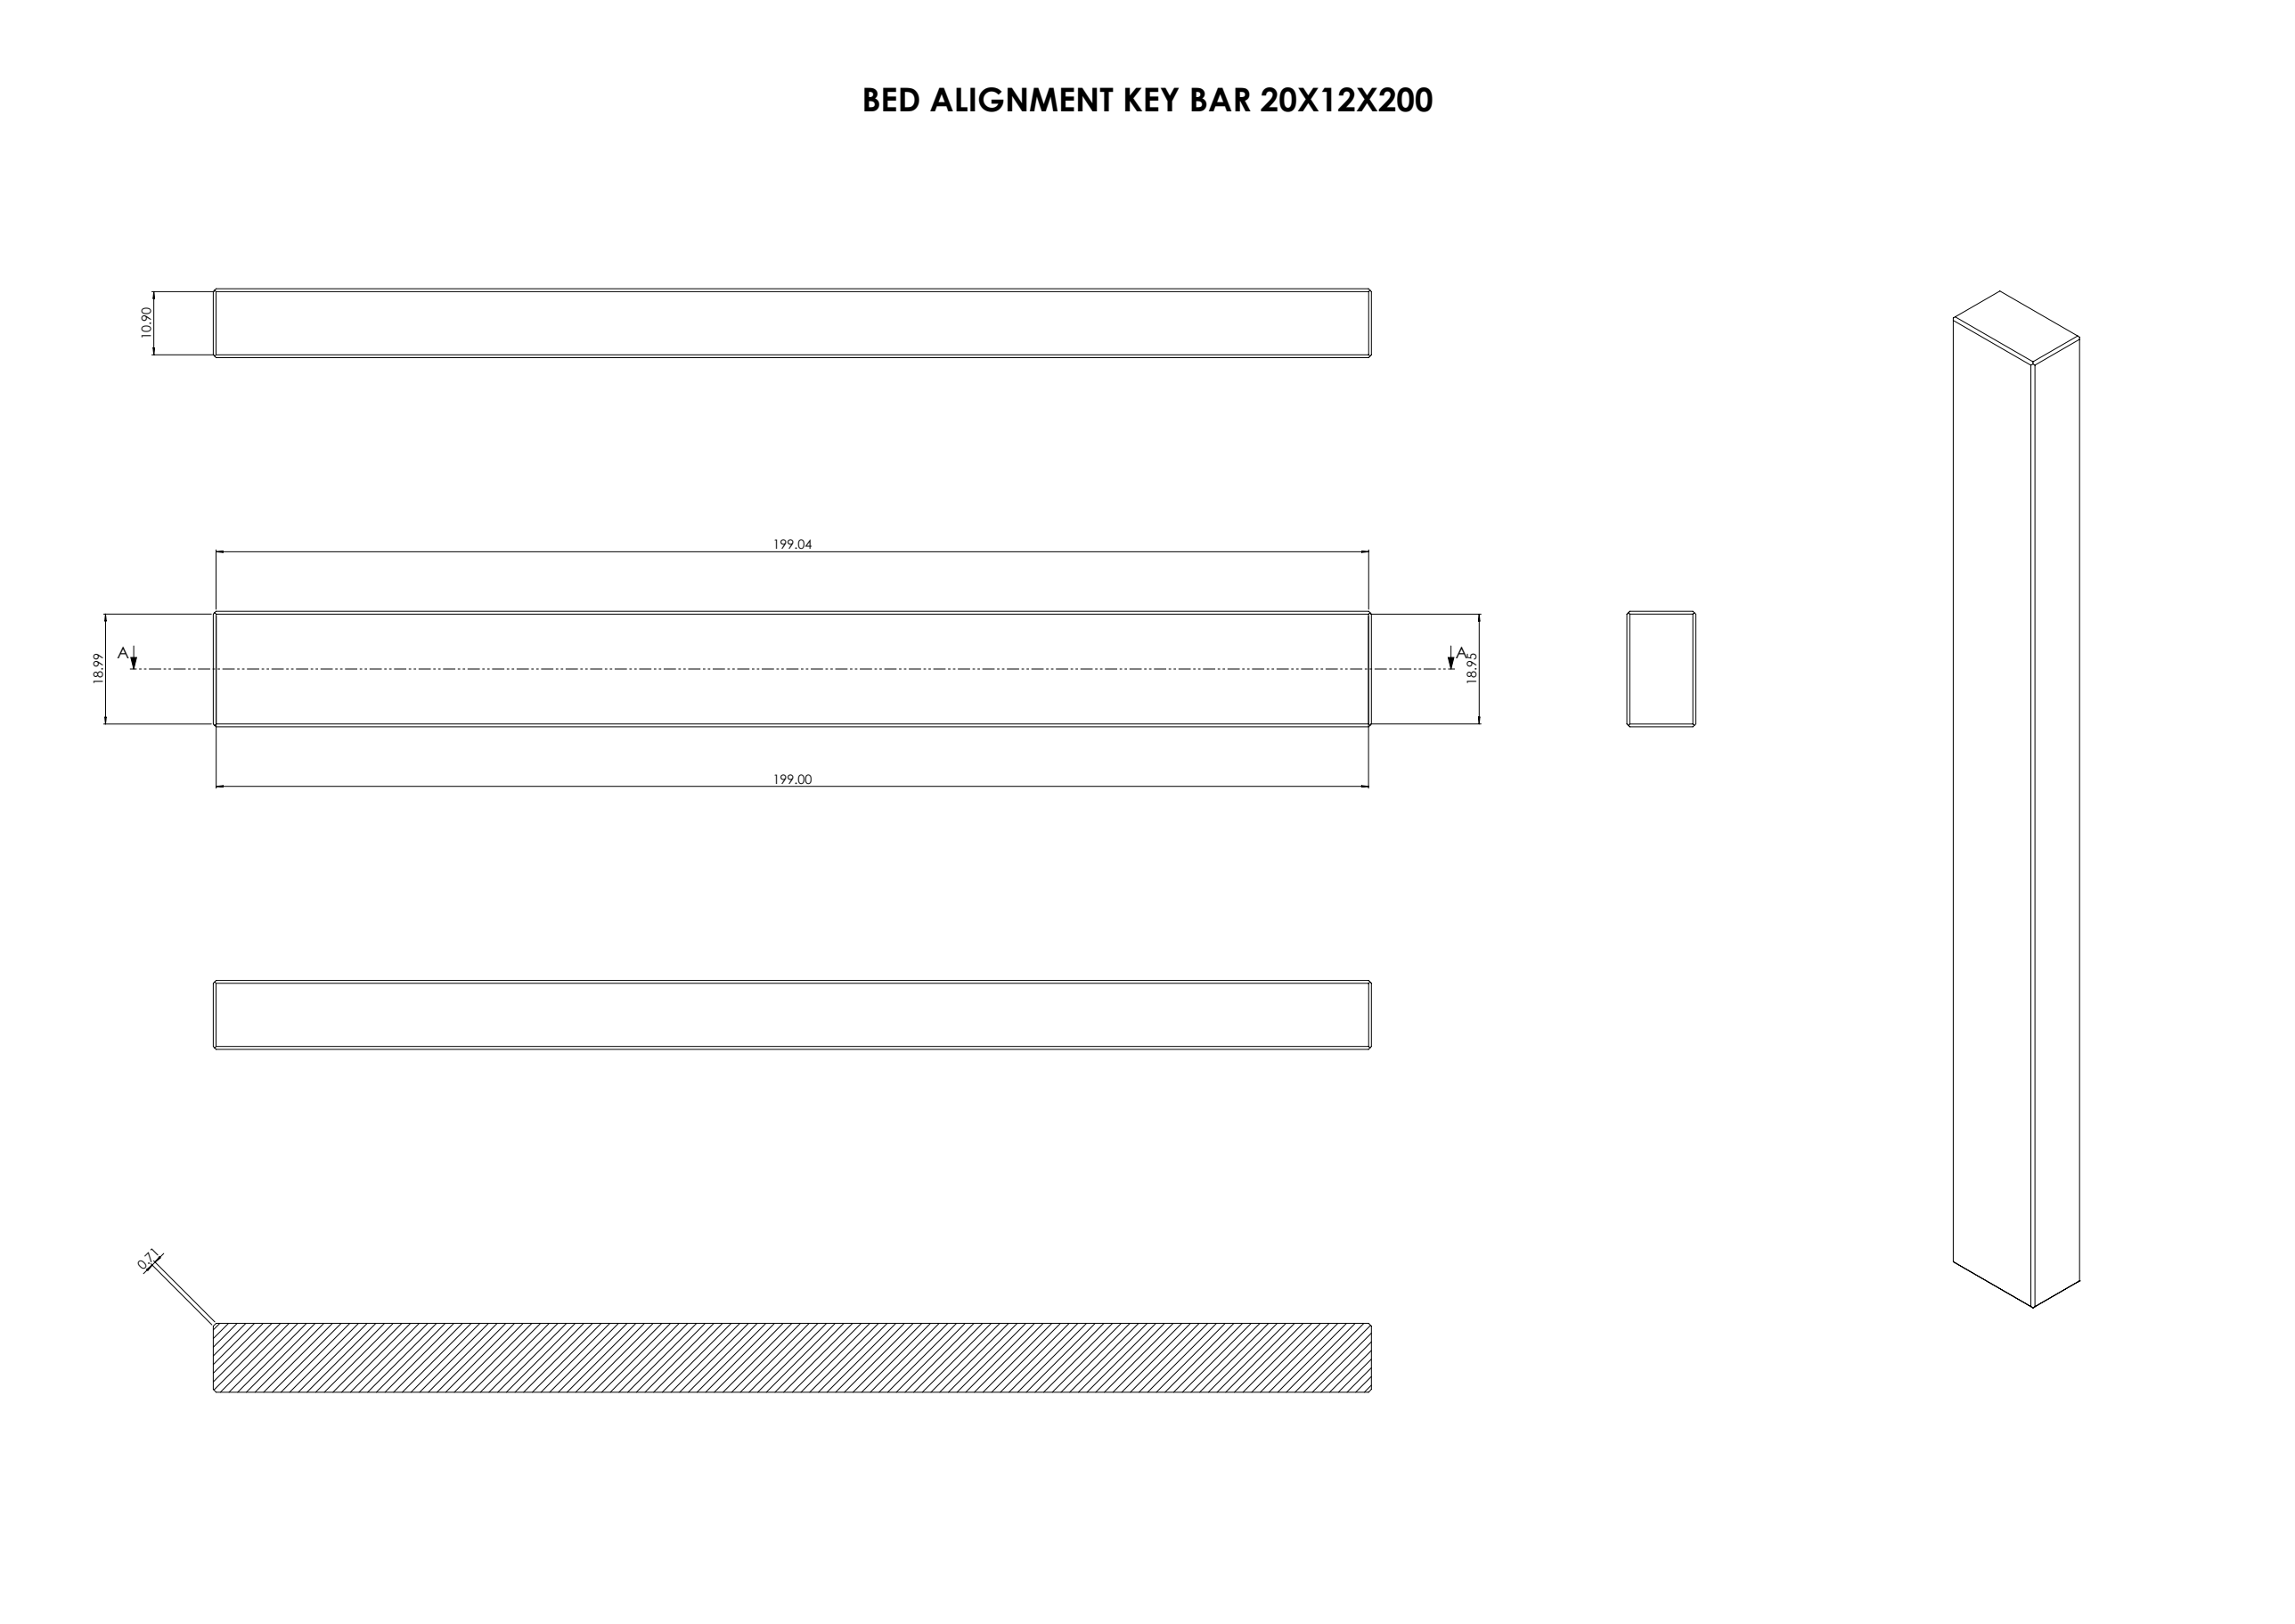
ISO-10303-21;
HEADER;
/* Generated by software containing ST-Developer
 * from STEP Tools, Inc. (www.steptools.com) 
 */

FILE_DESCRIPTION(
/* description */ (''),
/* implementation_level */ '2;1');

FILE_NAME(
/* name */ '16_Bed_Alignment_Key_Bar_20x12x200.step',
/* time_stamp */ '2026-10-26T03:50:32-07:00',
/* author */ (''),
/* organization */ (''),
/* preprocessor_version */ 'ST-DEVELOPER v20.2',
/* originating_system */ 'Autodesk Translation Framework v15.15.0.0',
/* authorisation */ '');

FILE_SCHEMA (('AUTOMOTIVE_DESIGN { 1 0 10303 214 3 1 1 }'));
ENDSEC;

DATA;
#10=MECHANICAL_DESIGN_GEOMETRIC_PRESENTATION_REPRESENTATION('',(#1052),#76660);
#1012=SHAPE_REPRESENTATION_RELATIONSHIP('SRR','None',#76749,#1032);
#1032=ADVANCED_BREP_SHAPE_REPRESENTATION('',(#1072),#76653);
#1052=STYLED_ITEM('',(#76906),#1072);
#1072=MANIFOLD_SOLID_BREP('Key bar',#26677);
#2130=PLANE('',#28345);
#2131=PLANE('',#28346);
#2132=PLANE('',#28347);
#2133=PLANE('',#28348);
#2134=PLANE('',#28349);
#2135=PLANE('',#28350);
#2136=PLANE('',#28351);
#2137=PLANE('',#28352);
#2138=PLANE('',#28353);
#2139=PLANE('',#28354);
#2140=PLANE('',#28355);
#2141=PLANE('',#28356);
#2142=PLANE('',#28357);
#2143=PLANE('',#28358);
#2144=PLANE('',#28359);
#2145=PLANE('',#28360);
#2146=PLANE('',#28361);
#2147=PLANE('',#28362);
#3436=FACE_OUTER_BOUND('',#5075,.T.);
#3437=FACE_OUTER_BOUND('',#5076,.T.);
#3438=FACE_OUTER_BOUND('',#5077,.T.);
#3439=FACE_OUTER_BOUND('',#5078,.T.);
#3440=FACE_OUTER_BOUND('',#5079,.T.);
#3441=FACE_OUTER_BOUND('',#5080,.T.);
#3442=FACE_OUTER_BOUND('',#5081,.T.);
#3443=FACE_OUTER_BOUND('',#5082,.T.);
#3444=FACE_OUTER_BOUND('',#5083,.T.);
#3445=FACE_OUTER_BOUND('',#5084,.T.);
#3446=FACE_OUTER_BOUND('',#5085,.T.);
#3447=FACE_OUTER_BOUND('',#5086,.T.);
#3448=FACE_OUTER_BOUND('',#5087,.T.);
#3449=FACE_OUTER_BOUND('',#5088,.T.);
#3450=FACE_OUTER_BOUND('',#5089,.T.);
#3451=FACE_OUTER_BOUND('',#5090,.T.);
#3452=FACE_OUTER_BOUND('',#5091,.T.);
#3453=FACE_OUTER_BOUND('',#5092,.T.);
#5075=EDGE_LOOP('',(#21705,#21706,#21707,#21708,#21709,#21710));
#5076=EDGE_LOOP('',(#21711,#21712,#21713,#21714));
#5077=EDGE_LOOP('',(#21715,#21716,#21717,#21718,#21719,#21720));
#5078=EDGE_LOOP('',(#21721,#21722,#21723,#21724,#21725,#21726));
#5079=EDGE_LOOP('',(#21727,#21728,#21729,#21730,#21731,#21732));
#5080=EDGE_LOOP('',(#21733,#21734,#21735,#21736,#21737,#21738));
#5081=EDGE_LOOP('',(#21739,#21740,#21741,#21742));
#5082=EDGE_LOOP('',(#21743,#21744,#21745,#21746,#21747,#21748));
#5083=EDGE_LOOP('',(#21749,#21750,#21751,#21752,#21753,#21754));
#5084=EDGE_LOOP('',(#21755,#21756,#21757,#21758));
#5085=EDGE_LOOP('',(#21759,#21760,#21761,#21762,#21763,#21764));
#5086=EDGE_LOOP('',(#21765,#21766,#21767,#21768,#21769,#21770));
#5087=EDGE_LOOP('',(#21771,#21772,#21773,#21774,#21775,#21776));
#5088=EDGE_LOOP('',(#21777,#21778,#21779,#21780,#21781,#21782));
#5089=EDGE_LOOP('',(#21783,#21784,#21785,#21786));
#5090=EDGE_LOOP('',(#21787,#21788,#21789,#21790,#21791,#21792));
#5091=EDGE_LOOP('',(#21793,#21794,#21795,#21796));
#5092=EDGE_LOOP('',(#21797,#21798,#21799,#21800));
#7856=LINE('',#58215,#10012);
#7857=LINE('',#58217,#10013);
#7858=LINE('',#58219,#10014);
#7859=LINE('',#58221,#10015);
#7860=LINE('',#58223,#10016);
#7861=LINE('',#58224,#10017);
#7862=LINE('',#58227,#10018);
#7863=LINE('',#58229,#10019);
#7864=LINE('',#58230,#10020);
#7865=LINE('',#58233,#10021);
#7866=LINE('',#58235,#10022);
#7867=LINE('',#58237,#10023);
#7868=LINE('',#58238,#10024);
#7869=LINE('',#58241,#10025);
#7870=LINE('',#58243,#10026);
#7871=LINE('',#58245,#10027);
#7872=LINE('',#58246,#10028);
#7873=LINE('',#58249,#10029);
#7874=LINE('',#58251,#10030);
#7875=LINE('',#58253,#10031);
#7876=LINE('',#58254,#10032);
#7877=LINE('',#58257,#10033);
#7878=LINE('',#58259,#10034);
#7879=LINE('',#58261,#10035);
#7880=LINE('',#58263,#10036);
#7881=LINE('',#58264,#10037);
#7882=LINE('',#58267,#10038);
#7883=LINE('',#58268,#10039);
#7884=LINE('',#58271,#10040);
#7885=LINE('',#58273,#10041);
#7886=LINE('',#58274,#10042);
#7887=LINE('',#58277,#10043);
#7888=LINE('',#58279,#10044);
#7889=LINE('',#58281,#10045);
#7890=LINE('',#58283,#10046);
#7891=LINE('',#58284,#10047);
#7892=LINE('',#58287,#10048);
#7893=LINE('',#58289,#10049);
#7894=LINE('',#58290,#10050);
#7895=LINE('',#58293,#10051);
#7896=LINE('',#58294,#10052);
#7897=LINE('',#58295,#10053);
#7898=LINE('',#58298,#10054);
#7899=LINE('',#58299,#10055);
#7900=LINE('',#58300,#10056);
#7901=LINE('',#58302,#10057);
#7902=LINE('',#58304,#10058);
#7903=LINE('',#58307,#10059);
#10012=VECTOR('',#33491,1.);
#10013=VECTOR('',#33492,1.);
#10014=VECTOR('',#33493,1.);
#10015=VECTOR('',#33494,1.);
#10016=VECTOR('',#33495,1.);
#10017=VECTOR('',#33496,1.);
#10018=VECTOR('',#33499,1.);
#10019=VECTOR('',#33500,1.);
#10020=VECTOR('',#33501,1.);
#10021=VECTOR('',#33504,1.);
#10022=VECTOR('',#33505,1.);
#10023=VECTOR('',#33506,1.);
#10024=VECTOR('',#33507,1.);
#10025=VECTOR('',#33510,1.);
#10026=VECTOR('',#33511,1.);
#10027=VECTOR('',#33512,1.);
#10028=VECTOR('',#33513,1.);
#10029=VECTOR('',#33516,1.);
#10030=VECTOR('',#33517,1.);
#10031=VECTOR('',#33518,1.);
#10032=VECTOR('',#33519,1.);
#10033=VECTOR('',#33522,1.);
#10034=VECTOR('',#33523,1.);
#10035=VECTOR('',#33524,1.);
#10036=VECTOR('',#33525,1.);
#10037=VECTOR('',#33526,1.);
#10038=VECTOR('',#33529,1.);
#10039=VECTOR('',#33530,1.);
#10040=VECTOR('',#33533,1.);
#10041=VECTOR('',#33534,1.);
#10042=VECTOR('',#33535,1.);
#10043=VECTOR('',#33538,1.);
#10044=VECTOR('',#33539,1.);
#10045=VECTOR('',#33540,1.);
#10046=VECTOR('',#33541,1.);
#10047=VECTOR('',#33542,1.);
#10048=VECTOR('',#33545,1.);
#10049=VECTOR('',#33546,1.);
#10050=VECTOR('',#33547,1.);
#10051=VECTOR('',#33550,1.);
#10052=VECTOR('',#33551,1.);
#10053=VECTOR('',#33552,1.);
#10054=VECTOR('',#33555,1.);
#10055=VECTOR('',#33556,1.);
#10056=VECTOR('',#33557,1.);
#10057=VECTOR('',#33560,1.);
#10058=VECTOR('',#33563,1.);
#10059=VECTOR('',#33568,1.);
#12319=VERTEX_POINT('',#58213);
#12320=VERTEX_POINT('',#58214);
#12321=VERTEX_POINT('',#58216);
#12322=VERTEX_POINT('',#58218);
#12323=VERTEX_POINT('',#58220);
#12324=VERTEX_POINT('',#58222);
#12325=VERTEX_POINT('',#58226);
#12326=VERTEX_POINT('',#58228);
#12327=VERTEX_POINT('',#58232);
#12328=VERTEX_POINT('',#58234);
#12329=VERTEX_POINT('',#58236);
#12330=VERTEX_POINT('',#58240);
#12331=VERTEX_POINT('',#58242);
#12332=VERTEX_POINT('',#58244);
#12333=VERTEX_POINT('',#58248);
#12334=VERTEX_POINT('',#58250);
#12335=VERTEX_POINT('',#58252);
#12336=VERTEX_POINT('',#58256);
#12337=VERTEX_POINT('',#58258);
#12338=VERTEX_POINT('',#58260);
#12339=VERTEX_POINT('',#58262);
#12340=VERTEX_POINT('',#58266);
#12341=VERTEX_POINT('',#58270);
#12342=VERTEX_POINT('',#58272);
#12343=VERTEX_POINT('',#58276);
#12344=VERTEX_POINT('',#58278);
#12345=VERTEX_POINT('',#58280);
#12346=VERTEX_POINT('',#58282);
#12347=VERTEX_POINT('',#58286);
#12348=VERTEX_POINT('',#58288);
#12349=VERTEX_POINT('',#58292);
#12350=VERTEX_POINT('',#58297);
#15575=EDGE_CURVE('',#12319,#12320,#7856,.T.);
#15576=EDGE_CURVE('',#12320,#12321,#7857,.T.);
#15577=EDGE_CURVE('',#12321,#12322,#7858,.T.);
#15578=EDGE_CURVE('',#12322,#12323,#7859,.T.);
#15579=EDGE_CURVE('',#12323,#12324,#7860,.T.);
#15580=EDGE_CURVE('',#12324,#12319,#7861,.T.);
#15581=EDGE_CURVE('',#12325,#12320,#7862,.T.);
#15582=EDGE_CURVE('',#12326,#12325,#7863,.T.);
#15583=EDGE_CURVE('',#12321,#12326,#7864,.T.);
#15584=EDGE_CURVE('',#12327,#12319,#7865,.T.);
#15585=EDGE_CURVE('',#12327,#12328,#7866,.T.);
#15586=EDGE_CURVE('',#12328,#12329,#7867,.T.);
#15587=EDGE_CURVE('',#12325,#12329,#7868,.T.);
#15588=EDGE_CURVE('',#12324,#12330,#7869,.T.);
#15589=EDGE_CURVE('',#12331,#12330,#7870,.T.);
#15590=EDGE_CURVE('',#12332,#12331,#7871,.T.);
#15591=EDGE_CURVE('',#12332,#12327,#7872,.T.);
#15592=EDGE_CURVE('',#12329,#12333,#7873,.T.);
#15593=EDGE_CURVE('',#12333,#12334,#7874,.T.);
#15594=EDGE_CURVE('',#12334,#12335,#7875,.T.);
#15595=EDGE_CURVE('',#12335,#12326,#7876,.T.);
#15596=EDGE_CURVE('',#12334,#12336,#7877,.T.);
#15597=EDGE_CURVE('',#12337,#12336,#7878,.T.);
#15598=EDGE_CURVE('',#12338,#12337,#7879,.T.);
#15599=EDGE_CURVE('',#12338,#12339,#7880,.T.);
#15600=EDGE_CURVE('',#12339,#12335,#7881,.T.);
#15601=EDGE_CURVE('',#12340,#12333,#7882,.T.);
#15602=EDGE_CURVE('',#12336,#12340,#7883,.T.);
#15603=EDGE_CURVE('',#12328,#12341,#7884,.T.);
#15604=EDGE_CURVE('',#12341,#12342,#7885,.T.);
#15605=EDGE_CURVE('',#12340,#12342,#7886,.T.);
#15606=EDGE_CURVE('',#12330,#12343,#7887,.T.);
#15607=EDGE_CURVE('',#12343,#12344,#7888,.T.);
#15608=EDGE_CURVE('',#12344,#12345,#7889,.T.);
#15609=EDGE_CURVE('',#12345,#12346,#7890,.T.);
#15610=EDGE_CURVE('',#12346,#12331,#7891,.T.);
#15611=EDGE_CURVE('',#12347,#12345,#7892,.T.);
#15612=EDGE_CURVE('',#12348,#12347,#7893,.T.);
#15613=EDGE_CURVE('',#12346,#12348,#7894,.T.);
#15614=EDGE_CURVE('',#12349,#12344,#7895,.T.);
#15615=EDGE_CURVE('',#12349,#12338,#7896,.T.);
#15616=EDGE_CURVE('',#12347,#12337,#7897,.T.);
#15617=EDGE_CURVE('',#12322,#12350,#7898,.T.);
#15618=EDGE_CURVE('',#12350,#12349,#7899,.T.);
#15619=EDGE_CURVE('',#12343,#12323,#7900,.T.);
#15620=EDGE_CURVE('',#12342,#12348,#7901,.T.);
#15621=EDGE_CURVE('',#12339,#12350,#7902,.T.);
#15622=EDGE_CURVE('',#12341,#12332,#7903,.T.);
#21705=ORIENTED_EDGE('',*,*,#15575,.T.);
#21706=ORIENTED_EDGE('',*,*,#15576,.T.);
#21707=ORIENTED_EDGE('',*,*,#15577,.T.);
#21708=ORIENTED_EDGE('',*,*,#15578,.T.);
#21709=ORIENTED_EDGE('',*,*,#15579,.T.);
#21710=ORIENTED_EDGE('',*,*,#15580,.T.);
#21711=ORIENTED_EDGE('',*,*,#15576,.F.);
#21712=ORIENTED_EDGE('',*,*,#15581,.F.);
#21713=ORIENTED_EDGE('',*,*,#15582,.F.);
#21714=ORIENTED_EDGE('',*,*,#15583,.F.);
#21715=ORIENTED_EDGE('',*,*,#15575,.F.);
#21716=ORIENTED_EDGE('',*,*,#15584,.F.);
#21717=ORIENTED_EDGE('',*,*,#15585,.T.);
#21718=ORIENTED_EDGE('',*,*,#15586,.T.);
#21719=ORIENTED_EDGE('',*,*,#15587,.F.);
#21720=ORIENTED_EDGE('',*,*,#15581,.T.);
#21721=ORIENTED_EDGE('',*,*,#15580,.F.);
#21722=ORIENTED_EDGE('',*,*,#15588,.T.);
#21723=ORIENTED_EDGE('',*,*,#15589,.F.);
#21724=ORIENTED_EDGE('',*,*,#15590,.F.);
#21725=ORIENTED_EDGE('',*,*,#15591,.T.);
#21726=ORIENTED_EDGE('',*,*,#15584,.T.);
#21727=ORIENTED_EDGE('',*,*,#15592,.T.);
#21728=ORIENTED_EDGE('',*,*,#15593,.T.);
#21729=ORIENTED_EDGE('',*,*,#15594,.T.);
#21730=ORIENTED_EDGE('',*,*,#15595,.T.);
#21731=ORIENTED_EDGE('',*,*,#15582,.T.);
#21732=ORIENTED_EDGE('',*,*,#15587,.T.);
#21733=ORIENTED_EDGE('',*,*,#15594,.F.);
#21734=ORIENTED_EDGE('',*,*,#15596,.T.);
#21735=ORIENTED_EDGE('',*,*,#15597,.F.);
#21736=ORIENTED_EDGE('',*,*,#15598,.F.);
#21737=ORIENTED_EDGE('',*,*,#15599,.T.);
#21738=ORIENTED_EDGE('',*,*,#15600,.T.);
#21739=ORIENTED_EDGE('',*,*,#15593,.F.);
#21740=ORIENTED_EDGE('',*,*,#15601,.F.);
#21741=ORIENTED_EDGE('',*,*,#15602,.F.);
#21742=ORIENTED_EDGE('',*,*,#15596,.F.);
#21743=ORIENTED_EDGE('',*,*,#15592,.F.);
#21744=ORIENTED_EDGE('',*,*,#15586,.F.);
#21745=ORIENTED_EDGE('',*,*,#15603,.T.);
#21746=ORIENTED_EDGE('',*,*,#15604,.T.);
#21747=ORIENTED_EDGE('',*,*,#15605,.F.);
#21748=ORIENTED_EDGE('',*,*,#15601,.T.);
#21749=ORIENTED_EDGE('',*,*,#15589,.T.);
#21750=ORIENTED_EDGE('',*,*,#15606,.T.);
#21751=ORIENTED_EDGE('',*,*,#15607,.T.);
#21752=ORIENTED_EDGE('',*,*,#15608,.T.);
#21753=ORIENTED_EDGE('',*,*,#15609,.T.);
#21754=ORIENTED_EDGE('',*,*,#15610,.T.);
#21755=ORIENTED_EDGE('',*,*,#15609,.F.);
#21756=ORIENTED_EDGE('',*,*,#15611,.F.);
#21757=ORIENTED_EDGE('',*,*,#15612,.F.);
#21758=ORIENTED_EDGE('',*,*,#15613,.F.);
#21759=ORIENTED_EDGE('',*,*,#15608,.F.);
#21760=ORIENTED_EDGE('',*,*,#15614,.F.);
#21761=ORIENTED_EDGE('',*,*,#15615,.T.);
#21762=ORIENTED_EDGE('',*,*,#15598,.T.);
#21763=ORIENTED_EDGE('',*,*,#15616,.F.);
#21764=ORIENTED_EDGE('',*,*,#15611,.T.);
#21765=ORIENTED_EDGE('',*,*,#15578,.F.);
#21766=ORIENTED_EDGE('',*,*,#15617,.T.);
#21767=ORIENTED_EDGE('',*,*,#15618,.T.);
#21768=ORIENTED_EDGE('',*,*,#15614,.T.);
#21769=ORIENTED_EDGE('',*,*,#15607,.F.);
#21770=ORIENTED_EDGE('',*,*,#15619,.T.);
#21771=ORIENTED_EDGE('',*,*,#15620,.T.);
#21772=ORIENTED_EDGE('',*,*,#15612,.T.);
#21773=ORIENTED_EDGE('',*,*,#15616,.T.);
#21774=ORIENTED_EDGE('',*,*,#15597,.T.);
#21775=ORIENTED_EDGE('',*,*,#15602,.T.);
#21776=ORIENTED_EDGE('',*,*,#15605,.T.);
#21777=ORIENTED_EDGE('',*,*,#15577,.F.);
#21778=ORIENTED_EDGE('',*,*,#15583,.T.);
#21779=ORIENTED_EDGE('',*,*,#15595,.F.);
#21780=ORIENTED_EDGE('',*,*,#15600,.F.);
#21781=ORIENTED_EDGE('',*,*,#15621,.T.);
#21782=ORIENTED_EDGE('',*,*,#15617,.F.);
#21783=ORIENTED_EDGE('',*,*,#15599,.F.);
#21784=ORIENTED_EDGE('',*,*,#15615,.F.);
#21785=ORIENTED_EDGE('',*,*,#15618,.F.);
#21786=ORIENTED_EDGE('',*,*,#15621,.F.);
#21787=ORIENTED_EDGE('',*,*,#15610,.F.);
#21788=ORIENTED_EDGE('',*,*,#15613,.T.);
#21789=ORIENTED_EDGE('',*,*,#15620,.F.);
#21790=ORIENTED_EDGE('',*,*,#15604,.F.);
#21791=ORIENTED_EDGE('',*,*,#15622,.T.);
#21792=ORIENTED_EDGE('',*,*,#15590,.T.);
#21793=ORIENTED_EDGE('',*,*,#15622,.F.);
#21794=ORIENTED_EDGE('',*,*,#15603,.F.);
#21795=ORIENTED_EDGE('',*,*,#15585,.F.);
#21796=ORIENTED_EDGE('',*,*,#15591,.F.);
#21797=ORIENTED_EDGE('',*,*,#15579,.F.);
#21798=ORIENTED_EDGE('',*,*,#15619,.F.);
#21799=ORIENTED_EDGE('',*,*,#15606,.F.);
#21800=ORIENTED_EDGE('',*,*,#15588,.F.);
#26024=ADVANCED_FACE('',(#3436),#2130,.T.);
#26025=ADVANCED_FACE('',(#3437),#2131,.T.);
#26026=ADVANCED_FACE('',(#3438),#2132,.T.);
#26027=ADVANCED_FACE('',(#3439),#2133,.T.);
#26028=ADVANCED_FACE('',(#3440),#2134,.T.);
#26029=ADVANCED_FACE('',(#3441),#2135,.T.);
#26030=ADVANCED_FACE('',(#3442),#2136,.T.);
#26031=ADVANCED_FACE('',(#3443),#2137,.T.);
#26032=ADVANCED_FACE('',(#3444),#2138,.T.);
#26033=ADVANCED_FACE('',(#3445),#2139,.T.);
#26034=ADVANCED_FACE('',(#3446),#2140,.T.);
#26035=ADVANCED_FACE('',(#3447),#2141,.T.);
#26036=ADVANCED_FACE('',(#3448),#2142,.T.);
#26037=ADVANCED_FACE('',(#3449),#2143,.T.);
#26038=ADVANCED_FACE('',(#3450),#2144,.F.);
#26039=ADVANCED_FACE('',(#3451),#2145,.T.);
#26040=ADVANCED_FACE('',(#3452),#2146,.T.);
#26041=ADVANCED_FACE('',(#3453),#2147,.T.);
#26677=CLOSED_SHELL('',(#26024,#26025,#26026,#26027,#26028,#26029,#26030,
#26031,#26032,#26033,#26034,#26035,#26036,#26037,#26038,#26039,#26040,#26041));
#28344=AXIS2_PLACEMENT_3D('',#58211,#33487,#33488);
#28345=AXIS2_PLACEMENT_3D('',#58212,#33489,#33490);
#28346=AXIS2_PLACEMENT_3D('',#58225,#33497,#33498);
#28347=AXIS2_PLACEMENT_3D('',#58231,#33502,#33503);
#28348=AXIS2_PLACEMENT_3D('',#58239,#33508,#33509);
#28349=AXIS2_PLACEMENT_3D('',#58247,#33514,#33515);
#28350=AXIS2_PLACEMENT_3D('',#58255,#33520,#33521);
#28351=AXIS2_PLACEMENT_3D('',#58265,#33527,#33528);
#28352=AXIS2_PLACEMENT_3D('',#58269,#33531,#33532);
#28353=AXIS2_PLACEMENT_3D('',#58275,#33536,#33537);
#28354=AXIS2_PLACEMENT_3D('',#58285,#33543,#33544);
#28355=AXIS2_PLACEMENT_3D('',#58291,#33548,#33549);
#28356=AXIS2_PLACEMENT_3D('',#58296,#33553,#33554);
#28357=AXIS2_PLACEMENT_3D('',#58301,#33558,#33559);
#28358=AXIS2_PLACEMENT_3D('',#58303,#33561,#33562);
#28359=AXIS2_PLACEMENT_3D('',#58305,#33564,#33565);
#28360=AXIS2_PLACEMENT_3D('',#58306,#33566,#33567);
#28361=AXIS2_PLACEMENT_3D('',#58308,#33569,#33570);
#28362=AXIS2_PLACEMENT_3D('',#58309,#33571,#33572);
#33487=DIRECTION('axis',(0.,0.,1.));
#33488=DIRECTION('refdir',(1.,0.,0.));
#33489=DIRECTION('center_axis',(-0.707106781186574,0.707106781186521,0.));
#33490=DIRECTION('ref_axis',(0.,0.,1.));
#33491=DIRECTION('',(0.577350269189601,0.577350269189643,-0.577350269189633));
#33492=DIRECTION('',(0.,0.,-1.));
#33493=DIRECTION('',(-0.577350269189601,-0.577350269189643,-0.577350269189633));
#33494=DIRECTION('',(-0.577350269189615,-0.577350269189658,0.577350269189605));
#33495=DIRECTION('',(0.,0.,1.));
#33496=DIRECTION('',(0.577350269189615,0.577350269189658,0.577350269189605));
#33497=DIRECTION('center_axis',(0.,1.,0.));
#33498=DIRECTION('ref_axis',(-1.,0.,0.));
#33499=DIRECTION('',(-1.,0.,0.));
#33500=DIRECTION('',(0.,0.,1.));
#33501=DIRECTION('',(1.,0.,0.));
#33502=DIRECTION('center_axis',(0.,0.707106781186541,0.707106781186554));
#33503=DIRECTION('ref_axis',(1.,0.,0.));
#33504=DIRECTION('',(-0.577350269189629,0.577350269189629,-0.577350269189619));
#33505=DIRECTION('',(1.,0.,0.));
#33506=DIRECTION('',(0.577350269189629,0.577350269189629,-0.577350269189619));
#33507=DIRECTION('',(0.577350269189601,-0.577350269189643,0.577350269189633));
#33508=DIRECTION('center_axis',(-0.707106781186541,0.,0.707106781186554));
#33509=DIRECTION('ref_axis',(0.707106781186554,0.,0.707106781186541));
#33510=DIRECTION('',(0.,-1.,0.));
#33511=DIRECTION('',(-0.577350269189615,0.577350269189658,-0.577350269189605));
#33512=DIRECTION('',(-0.577350269189629,-0.577350269189629,-0.577350269189619));
#33513=DIRECTION('',(0.,1.,0.));
#33514=DIRECTION('center_axis',(0.707106781186574,0.707106781186521,0.));
#33515=DIRECTION('ref_axis',(0.,0.,-1.));
#33516=DIRECTION('',(0.577350269189615,-0.577350269189658,-0.577350269189605));
#33517=DIRECTION('',(0.,0.,-1.));
#33518=DIRECTION('',(-0.577350269189615,0.577350269189658,-0.577350269189605));
#33519=DIRECTION('',(-0.577350269189601,0.577350269189643,0.577350269189633));
#33520=DIRECTION('center_axis',(0.707106781186541,0.,-0.707106781186554));
#33521=DIRECTION('ref_axis',(-0.707106781186554,0.,-0.707106781186541));
#33522=DIRECTION('',(0.,-1.,0.));
#33523=DIRECTION('',(0.577350269189615,0.577350269189658,0.577350269189605));
#33524=DIRECTION('',(0.577350269189629,-0.577350269189629,0.577350269189619));
#33525=DIRECTION('',(0.,1.,0.));
#33526=DIRECTION('',(0.577350269189629,0.577350269189629,0.577350269189619));
#33527=DIRECTION('center_axis',(1.,0.,0.));
#33528=DIRECTION('ref_axis',(0.,1.,0.));
#33529=DIRECTION('',(0.,1.,0.));
#33530=DIRECTION('',(0.,0.,1.));
#33531=DIRECTION('center_axis',(0.707106781186541,0.,0.707106781186554));
#33532=DIRECTION('ref_axis',(0.707106781186554,0.,-0.707106781186541));
#33533=DIRECTION('',(0.,-1.,0.));
#33534=DIRECTION('',(0.577350269189629,-0.577350269189629,-0.577350269189619));
#33535=DIRECTION('',(-0.577350269189615,-0.577350269189658,0.577350269189605));
#33536=DIRECTION('center_axis',(-0.707106781186574,-0.707106781186521,0.));
#33537=DIRECTION('ref_axis',(0.,0.,1.));
#33538=DIRECTION('',(0.,0.,-1.));
#33539=DIRECTION('',(0.577350269189615,-0.577350269189658,-0.577350269189605));
#33540=DIRECTION('',(0.577350269189601,-0.577350269189643,0.577350269189633));
#33541=DIRECTION('',(0.,0.,1.));
#33542=DIRECTION('',(-0.577350269189601,0.577350269189643,0.577350269189633));
#33543=DIRECTION('center_axis',(0.,-1.,0.));
#33544=DIRECTION('ref_axis',(1.,0.,0.));
#33545=DIRECTION('',(-1.,0.,0.));
#33546=DIRECTION('',(0.,0.,-1.));
#33547=DIRECTION('',(1.,0.,0.));
#33548=DIRECTION('center_axis',(0.,-0.707106781186541,-0.707106781186554));
#33549=DIRECTION('ref_axis',(-1.,0.,0.));
#33550=DIRECTION('',(-0.577350269189629,-0.577350269189629,0.577350269189619));
#33551=DIRECTION('',(1.,0.,0.));
#33552=DIRECTION('',(0.577350269189601,0.577350269189643,-0.577350269189633));
#33553=DIRECTION('center_axis',(-0.707106781186541,0.,-0.707106781186554));
#33554=DIRECTION('ref_axis',(-0.707106781186554,0.,0.707106781186541));
#33555=DIRECTION('',(0.577350269189629,-0.577350269189629,-0.577350269189619));
#33556=DIRECTION('',(0.,-1.,0.));
#33557=DIRECTION('',(0.,1.,0.));
#33558=DIRECTION('center_axis',(0.707106781186574,-0.707106781186521,0.));
#33559=DIRECTION('ref_axis',(0.,0.,-1.));
#33560=DIRECTION('',(-0.577350269189601,-0.577350269189643,-0.577350269189633));
#33561=DIRECTION('center_axis',(0.,0.707106781186541,-0.707106781186554));
#33562=DIRECTION('ref_axis',(-1.,0.,0.));
#33563=DIRECTION('',(-1.,0.,0.));
#33564=DIRECTION('center_axis',(0.,0.,1.));
#33565=DIRECTION('ref_axis',(1.,0.,0.));
#33566=DIRECTION('center_axis',(0.,-0.707106781186541,0.707106781186554));
#33567=DIRECTION('ref_axis',(1.,0.,0.));
#33568=DIRECTION('',(-1.,0.,0.));
#33569=DIRECTION('center_axis',(0.,0.,1.));
#33570=DIRECTION('ref_axis',(1.,0.,0.));
#33571=DIRECTION('center_axis',(-1.,0.,0.));
#33572=DIRECTION('ref_axis',(0.,-1.,0.));
#58211=CARTESIAN_POINT('',(0.,0.,0.));
#58212=CARTESIAN_POINT('Origin',(19.0265,9.976,3.6));
#58213=CARTESIAN_POINT('',(19.0265,9.976,4.764));
#58214=CARTESIAN_POINT('',(19.0505,10.,4.74));
#58215=CARTESIAN_POINT('',(19.4655416666666,10.4150416666667,4.32495833333334));
#58216=CARTESIAN_POINT('',(19.0505,10.,3.65));
#58217=CARTESIAN_POINT('',(19.0505,10.,3.6));
#58218=CARTESIAN_POINT('',(19.0265,9.976,3.626));
#58219=CARTESIAN_POINT('',(19.2672083333333,10.2167083333333,3.86670833333333));
#58220=CARTESIAN_POINT('',(19.0025,9.952,3.65));
#58221=CARTESIAN_POINT('',(18.2018333333333,9.15133333333324,4.45066666666668));
#58222=CARTESIAN_POINT('',(19.0025,9.952,4.74));
#58223=CARTESIAN_POINT('',(19.0025,9.952,3.6));
#58224=CARTESIAN_POINT('',(18.0035,8.95299999999991,3.741));
#58225=CARTESIAN_POINT('Origin',(20.9975,10.,3.6));
#58226=CARTESIAN_POINT('',(20.9495,10.,4.74));
#58227=CARTESIAN_POINT('',(20.49875,10.,4.74));
#58228=CARTESIAN_POINT('',(20.9495,10.,3.65));
#58229=CARTESIAN_POINT('',(20.9495,10.,3.6));
#58230=CARTESIAN_POINT('',(20.49875,10.,3.65));
#58231=CARTESIAN_POINT('Origin',(20.49875,9.975,4.765));
#58232=CARTESIAN_POINT('',(19.0525,9.95,4.79));
#58233=CARTESIAN_POINT('',(19.0525,9.95,4.79));
#58234=CARTESIAN_POINT('',(20.9475,9.95,4.79));
#58235=CARTESIAN_POINT('',(20.49875,9.95,4.79));
#58236=CARTESIAN_POINT('',(20.9735,9.976,4.764));
#58237=CARTESIAN_POINT('',(20.9475,9.95,4.79));
#58238=CARTESIAN_POINT('',(20.7007083333333,10.2487916666667,4.49120833333333));
#58239=CARTESIAN_POINT('Origin',(19.0275,5.,4.765));
#58240=CARTESIAN_POINT('',(19.0025,-9.952,4.74));
#58241=CARTESIAN_POINT('',(19.0025,5.,4.74));
#58242=CARTESIAN_POINT('',(19.0265,-9.976,4.764));
#58243=CARTESIAN_POINT('',(16.3368333333333,-7.28633333333305,2.0743333333333));
#58244=CARTESIAN_POINT('',(19.0525,-9.95,4.79));
#58245=CARTESIAN_POINT('',(19.0525,-9.95,4.79));
#58246=CARTESIAN_POINT('',(19.0525,5.,4.79));
#58247=CARTESIAN_POINT('Origin',(20.9735,9.976,3.6));
#58248=CARTESIAN_POINT('',(20.9975,9.952,4.74));
#58249=CARTESIAN_POINT('',(23.6631666666667,7.28633333333305,2.0743333333333));
#58250=CARTESIAN_POINT('',(20.9975,9.952,3.65));
#58251=CARTESIAN_POINT('',(20.9975,9.952,3.6));
#58252=CARTESIAN_POINT('',(20.9735,9.976,3.626));
#58253=CARTESIAN_POINT('',(23.4648333333334,7.48466666666639,6.11733333333338));
#58254=CARTESIAN_POINT('',(20.8990416666667,10.0504583333333,3.70045833333333));
#58255=CARTESIAN_POINT('Origin',(20.9725,-5.,3.625));
#58256=CARTESIAN_POINT('',(20.9975,-9.952,3.65));
#58257=CARTESIAN_POINT('',(20.9975,-5.,3.65));
#58258=CARTESIAN_POINT('',(20.9735,-9.976,3.626));
#58259=CARTESIAN_POINT('',(21.7981666666667,-9.15133333333324,4.45066666666668));
#58260=CARTESIAN_POINT('',(20.9475,-9.95,3.6));
#58261=CARTESIAN_POINT('',(20.9475,-9.95,3.6));
#58262=CARTESIAN_POINT('',(20.9475,9.95,3.6));
#58263=CARTESIAN_POINT('',(20.9475,-5.,3.6));
#58264=CARTESIAN_POINT('',(20.9475,9.95,3.6));
#58265=CARTESIAN_POINT('Origin',(20.9975,-10.,3.6));
#58266=CARTESIAN_POINT('',(20.9975,-9.952,4.74));
#58267=CARTESIAN_POINT('',(20.9975,-5.,4.74));
#58268=CARTESIAN_POINT('',(20.9975,-9.952,3.6));
#58269=CARTESIAN_POINT('Origin',(20.9725,-5.,4.765));
#58270=CARTESIAN_POINT('',(20.9475,-9.95,4.79));
#58271=CARTESIAN_POINT('',(20.9475,-5.,4.79));
#58272=CARTESIAN_POINT('',(20.9735,-9.976,4.764));
#58273=CARTESIAN_POINT('',(20.9475,-9.95,4.79));
#58274=CARTESIAN_POINT('',(21.9965,-8.95299999999991,3.741));
#58275=CARTESIAN_POINT('Origin',(19.0265,-9.976,3.6));
#58276=CARTESIAN_POINT('',(19.0025,-9.952,3.65));
#58277=CARTESIAN_POINT('',(19.0025,-9.952,3.6));
#58278=CARTESIAN_POINT('',(19.0265,-9.976,3.626));
#58279=CARTESIAN_POINT('',(16.5351666666666,-7.48466666666639,6.11733333333338));
#58280=CARTESIAN_POINT('',(19.0505,-10.,3.65));
#58281=CARTESIAN_POINT('',(19.1009583333333,-10.0504583333333,3.70045833333333));
#58282=CARTESIAN_POINT('',(19.0505,-10.,4.74));
#58283=CARTESIAN_POINT('',(19.0505,-10.,3.6));
#58284=CARTESIAN_POINT('',(19.2992916666667,-10.2487916666667,4.49120833333333));
#58285=CARTESIAN_POINT('Origin',(19.0025,-10.,3.6));
#58286=CARTESIAN_POINT('',(20.9495,-10.,3.65));
#58287=CARTESIAN_POINT('',(19.50125,-10.,3.65));
#58288=CARTESIAN_POINT('',(20.9495,-10.,4.74));
#58289=CARTESIAN_POINT('',(20.9495,-10.,3.6));
#58290=CARTESIAN_POINT('',(19.50125,-10.,4.74));
#58291=CARTESIAN_POINT('Origin',(19.50125,-9.975,3.625));
#58292=CARTESIAN_POINT('',(19.0525,-9.95,3.6));
#58293=CARTESIAN_POINT('',(19.0525,-9.95,3.6));
#58294=CARTESIAN_POINT('',(19.50125,-9.95,3.6));
#58295=CARTESIAN_POINT('',(20.7327916666667,-10.2167083333333,3.86670833333333));
#58296=CARTESIAN_POINT('Origin',(19.0275,5.,3.625));
#58297=CARTESIAN_POINT('',(19.0525,9.95,3.6));
#58298=CARTESIAN_POINT('',(19.0025,10.,3.65));
#58299=CARTESIAN_POINT('',(19.0525,5.,3.6));
#58300=CARTESIAN_POINT('',(19.0025,5.,3.65));
#58301=CARTESIAN_POINT('Origin',(20.9735,-9.976,3.6));
#58302=CARTESIAN_POINT('',(20.5344583333334,-10.4150416666667,4.32495833333334));
#58303=CARTESIAN_POINT('Origin',(20.49875,9.975,3.625));
#58304=CARTESIAN_POINT('',(20.49875,9.95,3.6));
#58305=CARTESIAN_POINT('Origin',(20.,0.,3.6));
#58306=CARTESIAN_POINT('Origin',(19.50125,-9.975,4.765));
#58307=CARTESIAN_POINT('',(19.50125,-9.95,4.79));
#58308=CARTESIAN_POINT('Origin',(20.,0.,4.79));
#58309=CARTESIAN_POINT('Origin',(19.0025,10.,3.6));
#76631=UNCERTAINTY_MEASURE_WITH_UNIT(LENGTH_MEASURE(0.001),#76661,
'DISTANCE_ACCURACY_VALUE',
'Maximum model space distance between geometric entities at asserted c
onnectivities');
#76638=UNCERTAINTY_MEASURE_WITH_UNIT(LENGTH_MEASURE(0.001),#76661,
'DISTANCE_ACCURACY_VALUE',
'Maximum model space distance between geometric entities at asserted c
onnectivities');
#76653=(
GEOMETRIC_REPRESENTATION_CONTEXT(3)
GLOBAL_UNCERTAINTY_ASSIGNED_CONTEXT((#76631))
GLOBAL_UNIT_ASSIGNED_CONTEXT((#76661,#76663,#76664))
REPRESENTATION_CONTEXT('','3D')
);
#76660=(
GEOMETRIC_REPRESENTATION_CONTEXT(3)
GLOBAL_UNCERTAINTY_ASSIGNED_CONTEXT((#76638))
GLOBAL_UNIT_ASSIGNED_CONTEXT((#76661,#76663,#76664))
REPRESENTATION_CONTEXT('','3D')
);
#76661=(
LENGTH_UNIT()
NAMED_UNIT(*)
SI_UNIT(.CENTI.,.METRE.)
);
#76663=(
NAMED_UNIT(*)
PLANE_ANGLE_UNIT()
SI_UNIT($,.RADIAN.)
);
#76664=(
NAMED_UNIT(*)
SI_UNIT($,.STERADIAN.)
SOLID_ANGLE_UNIT()
);
#76679=SHAPE_DEFINITION_REPRESENTATION(#76700,#76749);
#76700=PRODUCT_DEFINITION_SHAPE('',$,#76771);
#76749=SHAPE_REPRESENTATION('',(#28344),#76653);
#76756=PRODUCT_DEFINITION_CONTEXT('part definition',#76821,'design');
#76771=PRODUCT_DEFINITION('2026-10-26-11-13-33-347',
'16_Bed_Alignment_Key_Bar_20x12x200',#76792,#76756);
#76792=PRODUCT_DEFINITION_FORMATION('',$,#76837);
#76821=APPLICATION_CONTEXT(
'Core Data for Automotive Mechanical Design Process');
#76822=PRODUCT_CONTEXT('part definition',#76821,'mechanical');
#76837=PRODUCT('2026-10-26-11-13-33-347',
'16_Bed_Alignment_Key_Bar_20x12x200',$,(#76822));
#76900=COLOUR_RGB('Grey',0.48,0.52,0.57);
#76901=FILL_AREA_STYLE_COLOUR('',#76900);
#76902=FILL_AREA_STYLE('',(#76901));
#76903=SURFACE_STYLE_FILL_AREA(#76902);
#76904=SURFACE_SIDE_STYLE('',(#76903));
#76905=SURFACE_STYLE_USAGE(.BOTH.,#76904);
#76906=PRESENTATION_STYLE_ASSIGNMENT((#76905));
ENDSEC;
END-ISO-10303-21;
